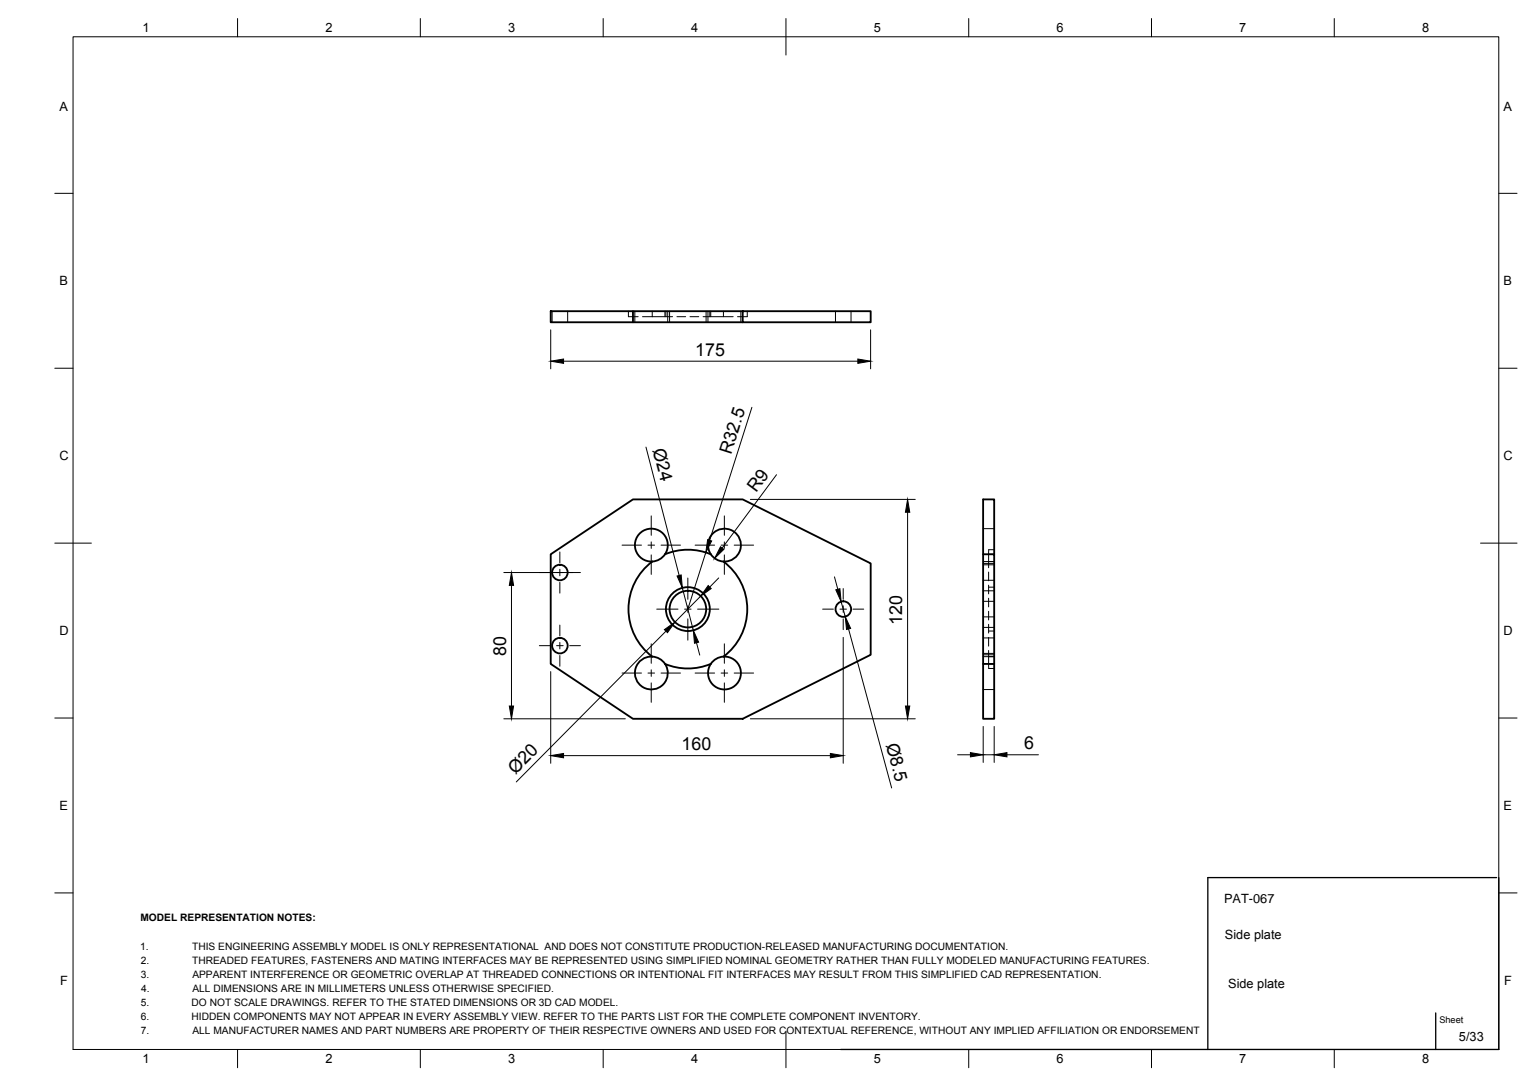
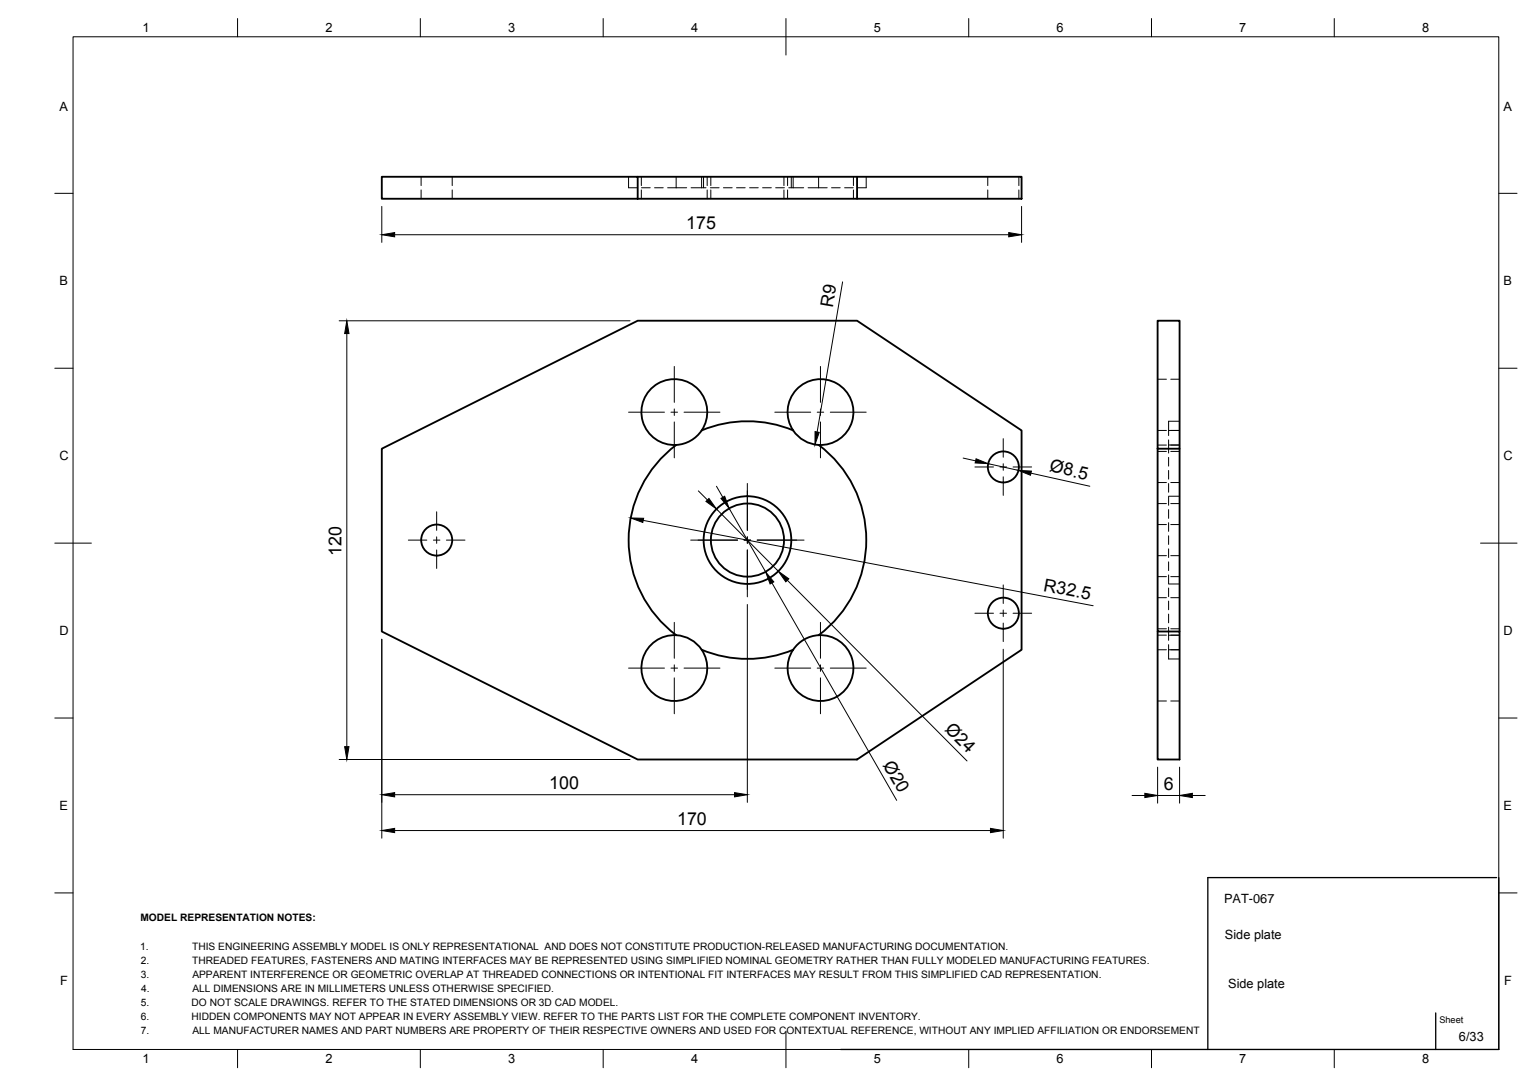
ISO-10303-21;
HEADER;
/* Generated by software containing ST-Developer
 * from STEP Tools, Inc. (www.steptools.com) 
 */

FILE_DESCRIPTION(
/* description */ ('Lifting hook block with sheave'),
/* implementation_level */ '2;1');

FILE_NAME(
/* name */ 'Side plate.step',
/* time_stamp */ '2026-10-28T03:23:54-07:00',
/* author */ (''),
/* organization */ (''),
/* preprocessor_version */ 'ST-DEVELOPER v20.2',
/* originating_system */ 'Autodesk Translation Framework v15.17.0.0',
/* authorisation */ '');

FILE_SCHEMA (('AUTOMOTIVE_DESIGN { 1 0 10303 214 3 1 1 }'));
ENDSEC;

DATA;
#10=MECHANICAL_DESIGN_GEOMETRIC_PRESENTATION_REPRESENTATION('',(#351),#9391);
#291=SHAPE_REPRESENTATION_RELATIONSHIP('SRR','None',#9522,#321);
#321=ADVANCED_BREP_SHAPE_REPRESENTATION('',(#389),#9357);
#351=STYLED_ITEM('',(#9752),#389);
#389=MANIFOLD_SOLID_BREP('Body1',#4887);
#424=LINE('',#7581,#712);
#425=LINE('',#7583,#713);
#426=LINE('',#7587,#714);
#427=LINE('',#7590,#715);
#428=LINE('',#7593,#716);
#429=LINE('',#7595,#717);
#430=LINE('',#7599,#718);
#431=LINE('',#7603,#719);
#432=LINE('',#7606,#720);
#433=LINE('',#7611,#721);
#434=LINE('',#7618,#722);
#435=LINE('',#7625,#723);
#436=LINE('',#7635,#724);
#437=LINE('',#7642,#725);
#438=LINE('',#7648,#726);
#439=LINE('',#7654,#727);
#440=LINE('',#7659,#728);
#441=LINE('',#7663,#729);
#442=LINE('',#7665,#730);
#443=LINE('',#7667,#731);
#444=LINE('',#7668,#732);
#445=LINE('',#7671,#733);
#446=LINE('',#7673,#734);
#447=LINE('',#7674,#735);
#448=LINE('',#7677,#736);
#449=LINE('',#7679,#737);
#450=LINE('',#7680,#738);
#451=LINE('',#7683,#739);
#452=LINE('',#7685,#740);
#453=LINE('',#7686,#741);
#454=LINE('',#7689,#742);
#455=LINE('',#7691,#743);
#456=LINE('',#7692,#744);
#457=LINE('',#7695,#745);
#458=LINE('',#7697,#746);
#459=LINE('',#7698,#747);
#460=LINE('',#7701,#748);
#461=LINE('',#7703,#749);
#462=LINE('',#7704,#750);
#463=LINE('',#7706,#751);
#464=LINE('',#7707,#752);
#712=VECTOR('',#5957,1.);
#713=VECTOR('',#5958,1.);
#714=VECTOR('',#5963,1.);
#715=VECTOR('',#5966,1.);
#716=VECTOR('',#5969,1.);
#717=VECTOR('',#5970,1.);
#718=VECTOR('',#5975,1.2);
#719=VECTOR('',#5980,1.);
#720=VECTOR('',#5983,1.);
#721=VECTOR('',#5988,0.9);
#722=VECTOR('',#5997,0.9);
#723=VECTOR('',#6006,0.9);
#724=VECTOR('',#6019,0.9);
#725=VECTOR('',#6028,0.425);
#726=VECTOR('',#6035,0.425);
#727=VECTOR('',#6042,0.425);
#728=VECTOR('',#6049,1.);
#729=VECTOR('',#6052,1.);
#730=VECTOR('',#6053,1.);
#731=VECTOR('',#6054,1.);
#732=VECTOR('',#6055,1.);
#733=VECTOR('',#6058,1.);
#734=VECTOR('',#6059,1.);
#735=VECTOR('',#6060,1.);
#736=VECTOR('',#6063,1.);
#737=VECTOR('',#6064,1.);
#738=VECTOR('',#6065,1.);
#739=VECTOR('',#6068,1.);
#740=VECTOR('',#6069,1.);
#741=VECTOR('',#6070,1.);
#742=VECTOR('',#6073,1.);
#743=VECTOR('',#6074,1.);
#744=VECTOR('',#6075,1.);
#745=VECTOR('',#6078,1.);
#746=VECTOR('',#6079,1.);
#747=VECTOR('',#6080,1.);
#748=VECTOR('',#6083,1.);
#749=VECTOR('',#6084,1.);
#750=VECTOR('',#6085,1.);
#751=VECTOR('',#6088,1.);
#752=VECTOR('',#6089,1.);
#1000=CYLINDRICAL_SURFACE('',#5272,3.25);
#1001=CYLINDRICAL_SURFACE('',#5274,3.25);
#1002=CYLINDRICAL_SURFACE('',#5276,3.25);
#1003=CYLINDRICAL_SURFACE('',#5278,1.2);
#1004=CYLINDRICAL_SURFACE('',#5280,3.25);
#1005=CYLINDRICAL_SURFACE('',#5282,0.9);
#1006=CYLINDRICAL_SURFACE('',#5286,0.9);
#1007=CYLINDRICAL_SURFACE('',#5290,0.9);
#1008=CYLINDRICAL_SURFACE('',#5296,0.9);
#1009=CYLINDRICAL_SURFACE('',#5300,0.425);
#1010=CYLINDRICAL_SURFACE('',#5303,0.425);
#1011=CYLINDRICAL_SURFACE('',#5306,0.425);
#1012=CYLINDRICAL_SURFACE('',#5309,1.);
#1107=FACE_BOUND('',#1512,.T.);
#1108=FACE_BOUND('',#1522,.T.);
#1109=FACE_BOUND('',#1537,.T.);
#1110=FACE_BOUND('',#1538,.T.);
#1111=FACE_BOUND('',#1539,.T.);
#1112=FACE_BOUND('',#1540,.T.);
#1113=FACE_BOUND('',#1542,.T.);
#1114=FACE_BOUND('',#1543,.T.);
#1115=FACE_BOUND('',#1544,.T.);
#1116=FACE_BOUND('',#1545,.T.);
#1117=FACE_BOUND('',#1546,.T.);
#1118=FACE_BOUND('',#1547,.T.);
#1119=FACE_BOUND('',#1548,.T.);
#1120=FACE_BOUND('',#1549,.T.);
#1222=FACE_OUTER_BOUND('',#1511,.T.);
#1223=FACE_OUTER_BOUND('',#1513,.T.);
#1224=FACE_OUTER_BOUND('',#1514,.T.);
#1225=FACE_OUTER_BOUND('',#1515,.T.);
#1226=FACE_OUTER_BOUND('',#1516,.T.);
#1227=FACE_OUTER_BOUND('',#1517,.T.);
#1228=FACE_OUTER_BOUND('',#1518,.T.);
#1229=FACE_OUTER_BOUND('',#1519,.T.);
#1230=FACE_OUTER_BOUND('',#1520,.T.);
#1231=FACE_OUTER_BOUND('',#1521,.T.);
#1232=FACE_OUTER_BOUND('',#1523,.T.);
#1233=FACE_OUTER_BOUND('',#1524,.T.);
#1234=FACE_OUTER_BOUND('',#1525,.T.);
#1235=FACE_OUTER_BOUND('',#1526,.T.);
#1236=FACE_OUTER_BOUND('',#1527,.T.);
#1237=FACE_OUTER_BOUND('',#1528,.T.);
#1238=FACE_OUTER_BOUND('',#1529,.T.);
#1239=FACE_OUTER_BOUND('',#1530,.T.);
#1240=FACE_OUTER_BOUND('',#1531,.T.);
#1241=FACE_OUTER_BOUND('',#1532,.T.);
#1242=FACE_OUTER_BOUND('',#1533,.T.);
#1243=FACE_OUTER_BOUND('',#1534,.T.);
#1244=FACE_OUTER_BOUND('',#1535,.T.);
#1245=FACE_OUTER_BOUND('',#1536,.T.);
#1246=FACE_OUTER_BOUND('',#1541,.T.);
#1511=EDGE_LOOP('',(#3230,#3231,#3232,#3233,#3234,#3235,#3236,#3237));
#1512=EDGE_LOOP('',(#3238));
#1513=EDGE_LOOP('',(#3239,#3240,#3241,#3242));
#1514=EDGE_LOOP('',(#3243,#3244,#3245,#3246));
#1515=EDGE_LOOP('',(#3247,#3248,#3249,#3250));
#1516=EDGE_LOOP('',(#3251,#3252,#3253,#3254));
#1517=EDGE_LOOP('',(#3255,#3256,#3257,#3258));
#1518=EDGE_LOOP('',(#3259,#3260,#3261,#3262,#3263,#3264,#3265,#3266));
#1519=EDGE_LOOP('',(#3267,#3268,#3269,#3270,#3271,#3272,#3273,#3274));
#1520=EDGE_LOOP('',(#3275,#3276,#3277,#3278,#3279,#3280,#3281,#3282));
#1521=EDGE_LOOP('',(#3283));
#1522=EDGE_LOOP('',(#3284));
#1523=EDGE_LOOP('',(#3285,#3286,#3287,#3288,#3289,#3290,#3291,#3292));
#1524=EDGE_LOOP('',(#3293,#3294,#3295,#3296));
#1525=EDGE_LOOP('',(#3297,#3298,#3299,#3300));
#1526=EDGE_LOOP('',(#3301,#3302,#3303,#3304));
#1527=EDGE_LOOP('',(#3305,#3306,#3307,#3308));
#1528=EDGE_LOOP('',(#3309,#3310,#3311,#3312));
#1529=EDGE_LOOP('',(#3313,#3314,#3315,#3316));
#1530=EDGE_LOOP('',(#3317,#3318,#3319,#3320));
#1531=EDGE_LOOP('',(#3321,#3322,#3323,#3324));
#1532=EDGE_LOOP('',(#3325,#3326,#3327,#3328));
#1533=EDGE_LOOP('',(#3329,#3330,#3331,#3332));
#1534=EDGE_LOOP('',(#3333,#3334,#3335,#3336));
#1535=EDGE_LOOP('',(#3337,#3338,#3339,#3340));
#1536=EDGE_LOOP('',(#3341,#3342,#3343,#3344,#3345,#3346,#3347,#3348));
#1537=EDGE_LOOP('',(#3349,#3350,#3351,#3352,#3353,#3354,#3355,#3356,#3357,
#3358,#3359,#3360));
#1538=EDGE_LOOP('',(#3361));
#1539=EDGE_LOOP('',(#3362));
#1540=EDGE_LOOP('',(#3363));
#1541=EDGE_LOOP('',(#3364,#3365,#3366,#3367,#3368,#3369,#3370,#3371));
#1542=EDGE_LOOP('',(#3372));
#1543=EDGE_LOOP('',(#3373));
#1544=EDGE_LOOP('',(#3374));
#1545=EDGE_LOOP('',(#3375));
#1546=EDGE_LOOP('',(#3376));
#1547=EDGE_LOOP('',(#3377));
#1548=EDGE_LOOP('',(#3378));
#1549=EDGE_LOOP('',(#3379));
#1915=CIRCLE('',#5263,0.9);
#1916=CIRCLE('',#5264,3.25);
#1917=CIRCLE('',#5265,0.9);
#1918=CIRCLE('',#5266,3.25);
#1919=CIRCLE('',#5267,0.9);
#1920=CIRCLE('',#5268,3.25);
#1921=CIRCLE('',#5269,0.9);
#1922=CIRCLE('',#5270,3.25);
#1923=CIRCLE('',#5271,1.2);
#1924=CIRCLE('',#5273,3.25);
#1925=CIRCLE('',#5275,3.25);
#1926=CIRCLE('',#5277,3.25);
#1927=CIRCLE('',#5279,1.2);
#1928=CIRCLE('',#5281,3.25);
#1929=CIRCLE('',#5283,0.9);
#1930=CIRCLE('',#5284,0.9);
#1931=CIRCLE('',#5285,0.9);
#1932=CIRCLE('',#5287,0.9);
#1933=CIRCLE('',#5288,0.9);
#1934=CIRCLE('',#5289,0.9);
#1935=CIRCLE('',#5291,0.9);
#1936=CIRCLE('',#5292,0.9);
#1937=CIRCLE('',#5293,0.9);
#1938=CIRCLE('',#5295,1.);
#1939=CIRCLE('',#5297,0.9);
#1940=CIRCLE('',#5298,0.9);
#1941=CIRCLE('',#5299,0.9);
#1942=CIRCLE('',#5301,0.425);
#1943=CIRCLE('',#5302,0.425);
#1944=CIRCLE('',#5304,0.425);
#1945=CIRCLE('',#5305,0.425);
#1946=CIRCLE('',#5307,0.425);
#1947=CIRCLE('',#5308,0.425);
#1948=CIRCLE('',#5310,1.);
#2208=VERTEX_POINT('',#7561);
#2209=VERTEX_POINT('',#7562);
#2210=VERTEX_POINT('',#7564);
#2211=VERTEX_POINT('',#7566);
#2212=VERTEX_POINT('',#7568);
#2213=VERTEX_POINT('',#7570);
#2214=VERTEX_POINT('',#7572);
#2215=VERTEX_POINT('',#7574);
#2216=VERTEX_POINT('',#7577);
#2217=VERTEX_POINT('',#7580);
#2218=VERTEX_POINT('',#7582);
#2219=VERTEX_POINT('',#7586);
#2220=VERTEX_POINT('',#7588);
#2221=VERTEX_POINT('',#7592);
#2222=VERTEX_POINT('',#7594);
#2223=VERTEX_POINT('',#7598);
#2224=VERTEX_POINT('',#7602);
#2225=VERTEX_POINT('',#7604);
#2226=VERTEX_POINT('',#7608);
#2227=VERTEX_POINT('',#7610);
#2228=VERTEX_POINT('',#7615);
#2229=VERTEX_POINT('',#7617);
#2230=VERTEX_POINT('',#7622);
#2231=VERTEX_POINT('',#7624);
#2232=VERTEX_POINT('',#7629);
#2233=VERTEX_POINT('',#7632);
#2234=VERTEX_POINT('',#7634);
#2235=VERTEX_POINT('',#7639);
#2236=VERTEX_POINT('',#7641);
#2237=VERTEX_POINT('',#7645);
#2238=VERTEX_POINT('',#7647);
#2239=VERTEX_POINT('',#7651);
#2240=VERTEX_POINT('',#7653);
#2241=VERTEX_POINT('',#7657);
#2242=VERTEX_POINT('',#7661);
#2243=VERTEX_POINT('',#7662);
#2244=VERTEX_POINT('',#7664);
#2245=VERTEX_POINT('',#7666);
#2246=VERTEX_POINT('',#7670);
#2247=VERTEX_POINT('',#7672);
#2248=VERTEX_POINT('',#7676);
#2249=VERTEX_POINT('',#7678);
#2250=VERTEX_POINT('',#7682);
#2251=VERTEX_POINT('',#7684);
#2252=VERTEX_POINT('',#7688);
#2253=VERTEX_POINT('',#7690);
#2254=VERTEX_POINT('',#7694);
#2255=VERTEX_POINT('',#7696);
#2256=VERTEX_POINT('',#7700);
#2257=VERTEX_POINT('',#7702);
#2619=EDGE_CURVE('',#2208,#2209,#1915,.T.);
#2620=EDGE_CURVE('',#2208,#2210,#1916,.T.);
#2621=EDGE_CURVE('',#2211,#2210,#1917,.T.);
#2622=EDGE_CURVE('',#2211,#2212,#1918,.T.);
#2623=EDGE_CURVE('',#2213,#2212,#1919,.T.);
#2624=EDGE_CURVE('',#2213,#2214,#1920,.T.);
#2625=EDGE_CURVE('',#2215,#2214,#1921,.T.);
#2626=EDGE_CURVE('',#2215,#2209,#1922,.T.);
#2627=EDGE_CURVE('',#2216,#2216,#1923,.T.);
#2628=EDGE_CURVE('',#2214,#2217,#424,.T.);
#2629=EDGE_CURVE('',#2218,#2213,#425,.T.);
#2630=EDGE_CURVE('',#2217,#2218,#1924,.T.);
#2631=EDGE_CURVE('',#2219,#2211,#426,.T.);
#2632=EDGE_CURVE('',#2220,#2219,#1925,.T.);
#2633=EDGE_CURVE('',#2212,#2220,#427,.T.);
#2634=EDGE_CURVE('',#2209,#2221,#428,.T.);
#2635=EDGE_CURVE('',#2222,#2215,#429,.T.);
#2636=EDGE_CURVE('',#2221,#2222,#1926,.T.);
#2637=EDGE_CURVE('',#2216,#2223,#430,.T.);
#2638=EDGE_CURVE('',#2223,#2223,#1927,.T.);
#2639=EDGE_CURVE('',#2224,#2208,#431,.T.);
#2640=EDGE_CURVE('',#2225,#2224,#1928,.T.);
#2641=EDGE_CURVE('',#2210,#2225,#432,.T.);
#2642=EDGE_CURVE('',#2226,#2226,#1929,.T.);
#2643=EDGE_CURVE('',#2226,#2227,#433,.T.);
#2644=EDGE_CURVE('',#2224,#2227,#1930,.T.);
#2645=EDGE_CURVE('',#2227,#2221,#1931,.T.);
#2646=EDGE_CURVE('',#2228,#2228,#1932,.T.);
#2647=EDGE_CURVE('',#2228,#2229,#434,.T.);
#2648=EDGE_CURVE('',#2222,#2229,#1933,.T.);
#2649=EDGE_CURVE('',#2229,#2217,#1934,.T.);
#2650=EDGE_CURVE('',#2230,#2230,#1935,.T.);
#2651=EDGE_CURVE('',#2230,#2231,#435,.T.);
#2652=EDGE_CURVE('',#2218,#2231,#1936,.T.);
#2653=EDGE_CURVE('',#2231,#2220,#1937,.T.);
#2654=EDGE_CURVE('',#2232,#2232,#1938,.T.);
#2655=EDGE_CURVE('',#2233,#2233,#1939,.T.);
#2656=EDGE_CURVE('',#2233,#2234,#436,.T.);
#2657=EDGE_CURVE('',#2219,#2234,#1940,.T.);
#2658=EDGE_CURVE('',#2234,#2225,#1941,.T.);
#2659=EDGE_CURVE('',#2235,#2235,#1942,.T.);
#2660=EDGE_CURVE('',#2235,#2236,#437,.T.);
#2661=EDGE_CURVE('',#2236,#2236,#1943,.T.);
#2662=EDGE_CURVE('',#2237,#2237,#1944,.T.);
#2663=EDGE_CURVE('',#2237,#2238,#438,.T.);
#2664=EDGE_CURVE('',#2238,#2238,#1945,.T.);
#2665=EDGE_CURVE('',#2239,#2239,#1946,.T.);
#2666=EDGE_CURVE('',#2239,#2240,#439,.T.);
#2667=EDGE_CURVE('',#2240,#2240,#1947,.T.);
#2668=EDGE_CURVE('',#2241,#2241,#1948,.T.);
#2669=EDGE_CURVE('',#2241,#2232,#440,.T.);
#2670=EDGE_CURVE('',#2242,#2243,#441,.T.);
#2671=EDGE_CURVE('',#2242,#2244,#442,.T.);
#2672=EDGE_CURVE('',#2245,#2244,#443,.T.);
#2673=EDGE_CURVE('',#2243,#2245,#444,.T.);
#2674=EDGE_CURVE('',#2243,#2246,#445,.T.);
#2675=EDGE_CURVE('',#2247,#2245,#446,.T.);
#2676=EDGE_CURVE('',#2246,#2247,#447,.T.);
#2677=EDGE_CURVE('',#2246,#2248,#448,.T.);
#2678=EDGE_CURVE('',#2249,#2247,#449,.T.);
#2679=EDGE_CURVE('',#2248,#2249,#450,.T.);
#2680=EDGE_CURVE('',#2248,#2250,#451,.T.);
#2681=EDGE_CURVE('',#2251,#2249,#452,.T.);
#2682=EDGE_CURVE('',#2250,#2251,#453,.T.);
#2683=EDGE_CURVE('',#2250,#2252,#454,.T.);
#2684=EDGE_CURVE('',#2253,#2251,#455,.T.);
#2685=EDGE_CURVE('',#2252,#2253,#456,.T.);
#2686=EDGE_CURVE('',#2252,#2254,#457,.T.);
#2687=EDGE_CURVE('',#2255,#2253,#458,.T.);
#2688=EDGE_CURVE('',#2254,#2255,#459,.T.);
#2689=EDGE_CURVE('',#2254,#2256,#460,.T.);
#2690=EDGE_CURVE('',#2257,#2255,#461,.T.);
#2691=EDGE_CURVE('',#2256,#2257,#462,.T.);
#2692=EDGE_CURVE('',#2256,#2242,#463,.T.);
#2693=EDGE_CURVE('',#2244,#2257,#464,.T.);
#3230=ORIENTED_EDGE('',*,*,#2619,.F.);
#3231=ORIENTED_EDGE('',*,*,#2620,.T.);
#3232=ORIENTED_EDGE('',*,*,#2621,.F.);
#3233=ORIENTED_EDGE('',*,*,#2622,.T.);
#3234=ORIENTED_EDGE('',*,*,#2623,.F.);
#3235=ORIENTED_EDGE('',*,*,#2624,.T.);
#3236=ORIENTED_EDGE('',*,*,#2625,.F.);
#3237=ORIENTED_EDGE('',*,*,#2626,.T.);
#3238=ORIENTED_EDGE('',*,*,#2627,.T.);
#3239=ORIENTED_EDGE('',*,*,#2628,.F.);
#3240=ORIENTED_EDGE('',*,*,#2624,.F.);
#3241=ORIENTED_EDGE('',*,*,#2629,.F.);
#3242=ORIENTED_EDGE('',*,*,#2630,.F.);
#3243=ORIENTED_EDGE('',*,*,#2631,.F.);
#3244=ORIENTED_EDGE('',*,*,#2632,.F.);
#3245=ORIENTED_EDGE('',*,*,#2633,.F.);
#3246=ORIENTED_EDGE('',*,*,#2622,.F.);
#3247=ORIENTED_EDGE('',*,*,#2634,.F.);
#3248=ORIENTED_EDGE('',*,*,#2626,.F.);
#3249=ORIENTED_EDGE('',*,*,#2635,.F.);
#3250=ORIENTED_EDGE('',*,*,#2636,.F.);
#3251=ORIENTED_EDGE('',*,*,#2627,.F.);
#3252=ORIENTED_EDGE('',*,*,#2637,.T.);
#3253=ORIENTED_EDGE('',*,*,#2638,.F.);
#3254=ORIENTED_EDGE('',*,*,#2637,.F.);
#3255=ORIENTED_EDGE('',*,*,#2639,.F.);
#3256=ORIENTED_EDGE('',*,*,#2640,.F.);
#3257=ORIENTED_EDGE('',*,*,#2641,.F.);
#3258=ORIENTED_EDGE('',*,*,#2620,.F.);
#3259=ORIENTED_EDGE('',*,*,#2642,.F.);
#3260=ORIENTED_EDGE('',*,*,#2643,.T.);
#3261=ORIENTED_EDGE('',*,*,#2644,.F.);
#3262=ORIENTED_EDGE('',*,*,#2639,.T.);
#3263=ORIENTED_EDGE('',*,*,#2619,.T.);
#3264=ORIENTED_EDGE('',*,*,#2634,.T.);
#3265=ORIENTED_EDGE('',*,*,#2645,.F.);
#3266=ORIENTED_EDGE('',*,*,#2643,.F.);
#3267=ORIENTED_EDGE('',*,*,#2646,.F.);
#3268=ORIENTED_EDGE('',*,*,#2647,.T.);
#3269=ORIENTED_EDGE('',*,*,#2648,.F.);
#3270=ORIENTED_EDGE('',*,*,#2635,.T.);
#3271=ORIENTED_EDGE('',*,*,#2625,.T.);
#3272=ORIENTED_EDGE('',*,*,#2628,.T.);
#3273=ORIENTED_EDGE('',*,*,#2649,.F.);
#3274=ORIENTED_EDGE('',*,*,#2647,.F.);
#3275=ORIENTED_EDGE('',*,*,#2650,.F.);
#3276=ORIENTED_EDGE('',*,*,#2651,.T.);
#3277=ORIENTED_EDGE('',*,*,#2652,.F.);
#3278=ORIENTED_EDGE('',*,*,#2629,.T.);
#3279=ORIENTED_EDGE('',*,*,#2623,.T.);
#3280=ORIENTED_EDGE('',*,*,#2633,.T.);
#3281=ORIENTED_EDGE('',*,*,#2653,.F.);
#3282=ORIENTED_EDGE('',*,*,#2651,.F.);
#3283=ORIENTED_EDGE('',*,*,#2638,.T.);
#3284=ORIENTED_EDGE('',*,*,#2654,.T.);
#3285=ORIENTED_EDGE('',*,*,#2655,.F.);
#3286=ORIENTED_EDGE('',*,*,#2656,.T.);
#3287=ORIENTED_EDGE('',*,*,#2657,.F.);
#3288=ORIENTED_EDGE('',*,*,#2631,.T.);
#3289=ORIENTED_EDGE('',*,*,#2621,.T.);
#3290=ORIENTED_EDGE('',*,*,#2641,.T.);
#3291=ORIENTED_EDGE('',*,*,#2658,.F.);
#3292=ORIENTED_EDGE('',*,*,#2656,.F.);
#3293=ORIENTED_EDGE('',*,*,#2659,.F.);
#3294=ORIENTED_EDGE('',*,*,#2660,.T.);
#3295=ORIENTED_EDGE('',*,*,#2661,.F.);
#3296=ORIENTED_EDGE('',*,*,#2660,.F.);
#3297=ORIENTED_EDGE('',*,*,#2662,.F.);
#3298=ORIENTED_EDGE('',*,*,#2663,.T.);
#3299=ORIENTED_EDGE('',*,*,#2664,.F.);
#3300=ORIENTED_EDGE('',*,*,#2663,.F.);
#3301=ORIENTED_EDGE('',*,*,#2665,.F.);
#3302=ORIENTED_EDGE('',*,*,#2666,.T.);
#3303=ORIENTED_EDGE('',*,*,#2667,.F.);
#3304=ORIENTED_EDGE('',*,*,#2666,.F.);
#3305=ORIENTED_EDGE('',*,*,#2668,.F.);
#3306=ORIENTED_EDGE('',*,*,#2669,.T.);
#3307=ORIENTED_EDGE('',*,*,#2654,.F.);
#3308=ORIENTED_EDGE('',*,*,#2669,.F.);
#3309=ORIENTED_EDGE('',*,*,#2670,.F.);
#3310=ORIENTED_EDGE('',*,*,#2671,.T.);
#3311=ORIENTED_EDGE('',*,*,#2672,.F.);
#3312=ORIENTED_EDGE('',*,*,#2673,.F.);
#3313=ORIENTED_EDGE('',*,*,#2674,.F.);
#3314=ORIENTED_EDGE('',*,*,#2673,.T.);
#3315=ORIENTED_EDGE('',*,*,#2675,.F.);
#3316=ORIENTED_EDGE('',*,*,#2676,.F.);
#3317=ORIENTED_EDGE('',*,*,#2677,.F.);
#3318=ORIENTED_EDGE('',*,*,#2676,.T.);
#3319=ORIENTED_EDGE('',*,*,#2678,.F.);
#3320=ORIENTED_EDGE('',*,*,#2679,.F.);
#3321=ORIENTED_EDGE('',*,*,#2680,.F.);
#3322=ORIENTED_EDGE('',*,*,#2679,.T.);
#3323=ORIENTED_EDGE('',*,*,#2681,.F.);
#3324=ORIENTED_EDGE('',*,*,#2682,.F.);
#3325=ORIENTED_EDGE('',*,*,#2683,.F.);
#3326=ORIENTED_EDGE('',*,*,#2682,.T.);
#3327=ORIENTED_EDGE('',*,*,#2684,.F.);
#3328=ORIENTED_EDGE('',*,*,#2685,.F.);
#3329=ORIENTED_EDGE('',*,*,#2686,.F.);
#3330=ORIENTED_EDGE('',*,*,#2685,.T.);
#3331=ORIENTED_EDGE('',*,*,#2687,.F.);
#3332=ORIENTED_EDGE('',*,*,#2688,.F.);
#3333=ORIENTED_EDGE('',*,*,#2689,.F.);
#3334=ORIENTED_EDGE('',*,*,#2688,.T.);
#3335=ORIENTED_EDGE('',*,*,#2690,.F.);
#3336=ORIENTED_EDGE('',*,*,#2691,.F.);
#3337=ORIENTED_EDGE('',*,*,#2692,.F.);
#3338=ORIENTED_EDGE('',*,*,#2691,.T.);
#3339=ORIENTED_EDGE('',*,*,#2693,.F.);
#3340=ORIENTED_EDGE('',*,*,#2671,.F.);
#3341=ORIENTED_EDGE('',*,*,#2693,.T.);
#3342=ORIENTED_EDGE('',*,*,#2690,.T.);
#3343=ORIENTED_EDGE('',*,*,#2687,.T.);
#3344=ORIENTED_EDGE('',*,*,#2684,.T.);
#3345=ORIENTED_EDGE('',*,*,#2681,.T.);
#3346=ORIENTED_EDGE('',*,*,#2678,.T.);
#3347=ORIENTED_EDGE('',*,*,#2675,.T.);
#3348=ORIENTED_EDGE('',*,*,#2672,.T.);
#3349=ORIENTED_EDGE('',*,*,#2640,.T.);
#3350=ORIENTED_EDGE('',*,*,#2644,.T.);
#3351=ORIENTED_EDGE('',*,*,#2645,.T.);
#3352=ORIENTED_EDGE('',*,*,#2636,.T.);
#3353=ORIENTED_EDGE('',*,*,#2648,.T.);
#3354=ORIENTED_EDGE('',*,*,#2649,.T.);
#3355=ORIENTED_EDGE('',*,*,#2630,.T.);
#3356=ORIENTED_EDGE('',*,*,#2652,.T.);
#3357=ORIENTED_EDGE('',*,*,#2653,.T.);
#3358=ORIENTED_EDGE('',*,*,#2632,.T.);
#3359=ORIENTED_EDGE('',*,*,#2657,.T.);
#3360=ORIENTED_EDGE('',*,*,#2658,.T.);
#3361=ORIENTED_EDGE('',*,*,#2667,.T.);
#3362=ORIENTED_EDGE('',*,*,#2664,.T.);
#3363=ORIENTED_EDGE('',*,*,#2661,.T.);
#3364=ORIENTED_EDGE('',*,*,#2692,.T.);
#3365=ORIENTED_EDGE('',*,*,#2670,.T.);
#3366=ORIENTED_EDGE('',*,*,#2674,.T.);
#3367=ORIENTED_EDGE('',*,*,#2677,.T.);
#3368=ORIENTED_EDGE('',*,*,#2680,.T.);
#3369=ORIENTED_EDGE('',*,*,#2683,.T.);
#3370=ORIENTED_EDGE('',*,*,#2686,.T.);
#3371=ORIENTED_EDGE('',*,*,#2689,.T.);
#3372=ORIENTED_EDGE('',*,*,#2668,.T.);
#3373=ORIENTED_EDGE('',*,*,#2665,.T.);
#3374=ORIENTED_EDGE('',*,*,#2662,.T.);
#3375=ORIENTED_EDGE('',*,*,#2659,.T.);
#3376=ORIENTED_EDGE('',*,*,#2650,.T.);
#3377=ORIENTED_EDGE('',*,*,#2642,.T.);
#3378=ORIENTED_EDGE('',*,*,#2655,.T.);
#3379=ORIENTED_EDGE('',*,*,#2646,.T.);
#4452=PLANE('',#5262);
#4453=PLANE('',#5294);
#4454=PLANE('',#5311);
#4455=PLANE('',#5312);
#4456=PLANE('',#5313);
#4457=PLANE('',#5314);
#4458=PLANE('',#5315);
#4459=PLANE('',#5316);
#4460=PLANE('',#5317);
#4461=PLANE('',#5318);
#4462=PLANE('',#5319);
#4463=PLANE('',#5320);
#4598=ADVANCED_FACE('',(#1222,#1107),#4452,.T.);
#4599=ADVANCED_FACE('',(#1223),#1000,.F.);
#4600=ADVANCED_FACE('',(#1224),#1001,.F.);
#4601=ADVANCED_FACE('',(#1225),#1002,.F.);
#4602=ADVANCED_FACE('',(#1226),#1003,.T.);
#4603=ADVANCED_FACE('',(#1227),#1004,.F.);
#4604=ADVANCED_FACE('',(#1228),#1005,.F.);
#4605=ADVANCED_FACE('',(#1229),#1006,.F.);
#4606=ADVANCED_FACE('',(#1230),#1007,.F.);
#4607=ADVANCED_FACE('',(#1231,#1108),#4453,.T.);
#4608=ADVANCED_FACE('',(#1232),#1008,.F.);
#4609=ADVANCED_FACE('',(#1233),#1009,.F.);
#4610=ADVANCED_FACE('',(#1234),#1010,.F.);
#4611=ADVANCED_FACE('',(#1235),#1011,.F.);
#4612=ADVANCED_FACE('',(#1236),#1012,.F.);
#4613=ADVANCED_FACE('',(#1237),#4454,.T.);
#4614=ADVANCED_FACE('',(#1238),#4455,.T.);
#4615=ADVANCED_FACE('',(#1239),#4456,.T.);
#4616=ADVANCED_FACE('',(#1240),#4457,.T.);
#4617=ADVANCED_FACE('',(#1241),#4458,.T.);
#4618=ADVANCED_FACE('',(#1242),#4459,.T.);
#4619=ADVANCED_FACE('',(#1243),#4460,.T.);
#4620=ADVANCED_FACE('',(#1244),#4461,.T.);
#4621=ADVANCED_FACE('',(#1245,#1109,#1110,#1111,#1112),#4462,.T.);
#4622=ADVANCED_FACE('',(#1246,#1113,#1114,#1115,#1116,#1117,#1118,#1119,
#1120),#4463,.F.);
#4887=CLOSED_SHELL('',(#4598,#4599,#4600,#4601,#4602,#4603,#4604,#4605,
#4606,#4607,#4608,#4609,#4610,#4611,#4612,#4613,#4614,#4615,#4616,#4617,
#4618,#4619,#4620,#4621,#4622));
#5261=AXIS2_PLACEMENT_3D('',#7559,#5933,#5934);
#5262=AXIS2_PLACEMENT_3D('',#7560,#5935,#5936);
#5263=AXIS2_PLACEMENT_3D('',#7563,#5937,#5938);
#5264=AXIS2_PLACEMENT_3D('',#7565,#5939,#5940);
#5265=AXIS2_PLACEMENT_3D('',#7567,#5941,#5942);
#5266=AXIS2_PLACEMENT_3D('',#7569,#5943,#5944);
#5267=AXIS2_PLACEMENT_3D('',#7571,#5945,#5946);
#5268=AXIS2_PLACEMENT_3D('',#7573,#5947,#5948);
#5269=AXIS2_PLACEMENT_3D('',#7575,#5949,#5950);
#5270=AXIS2_PLACEMENT_3D('',#7576,#5951,#5952);
#5271=AXIS2_PLACEMENT_3D('',#7578,#5953,#5954);
#5272=AXIS2_PLACEMENT_3D('',#7579,#5955,#5956);
#5273=AXIS2_PLACEMENT_3D('',#7584,#5959,#5960);
#5274=AXIS2_PLACEMENT_3D('',#7585,#5961,#5962);
#5275=AXIS2_PLACEMENT_3D('',#7589,#5964,#5965);
#5276=AXIS2_PLACEMENT_3D('',#7591,#5967,#5968);
#5277=AXIS2_PLACEMENT_3D('',#7596,#5971,#5972);
#5278=AXIS2_PLACEMENT_3D('',#7597,#5973,#5974);
#5279=AXIS2_PLACEMENT_3D('',#7600,#5976,#5977);
#5280=AXIS2_PLACEMENT_3D('',#7601,#5978,#5979);
#5281=AXIS2_PLACEMENT_3D('',#7605,#5981,#5982);
#5282=AXIS2_PLACEMENT_3D('',#7607,#5984,#5985);
#5283=AXIS2_PLACEMENT_3D('',#7609,#5986,#5987);
#5284=AXIS2_PLACEMENT_3D('',#7612,#5989,#5990);
#5285=AXIS2_PLACEMENT_3D('',#7613,#5991,#5992);
#5286=AXIS2_PLACEMENT_3D('',#7614,#5993,#5994);
#5287=AXIS2_PLACEMENT_3D('',#7616,#5995,#5996);
#5288=AXIS2_PLACEMENT_3D('',#7619,#5998,#5999);
#5289=AXIS2_PLACEMENT_3D('',#7620,#6000,#6001);
#5290=AXIS2_PLACEMENT_3D('',#7621,#6002,#6003);
#5291=AXIS2_PLACEMENT_3D('',#7623,#6004,#6005);
#5292=AXIS2_PLACEMENT_3D('',#7626,#6007,#6008);
#5293=AXIS2_PLACEMENT_3D('',#7627,#6009,#6010);
#5294=AXIS2_PLACEMENT_3D('',#7628,#6011,#6012);
#5295=AXIS2_PLACEMENT_3D('',#7630,#6013,#6014);
#5296=AXIS2_PLACEMENT_3D('',#7631,#6015,#6016);
#5297=AXIS2_PLACEMENT_3D('',#7633,#6017,#6018);
#5298=AXIS2_PLACEMENT_3D('',#7636,#6020,#6021);
#5299=AXIS2_PLACEMENT_3D('',#7637,#6022,#6023);
#5300=AXIS2_PLACEMENT_3D('',#7638,#6024,#6025);
#5301=AXIS2_PLACEMENT_3D('',#7640,#6026,#6027);
#5302=AXIS2_PLACEMENT_3D('',#7643,#6029,#6030);
#5303=AXIS2_PLACEMENT_3D('',#7644,#6031,#6032);
#5304=AXIS2_PLACEMENT_3D('',#7646,#6033,#6034);
#5305=AXIS2_PLACEMENT_3D('',#7649,#6036,#6037);
#5306=AXIS2_PLACEMENT_3D('',#7650,#6038,#6039);
#5307=AXIS2_PLACEMENT_3D('',#7652,#6040,#6041);
#5308=AXIS2_PLACEMENT_3D('',#7655,#6043,#6044);
#5309=AXIS2_PLACEMENT_3D('',#7656,#6045,#6046);
#5310=AXIS2_PLACEMENT_3D('',#7658,#6047,#6048);
#5311=AXIS2_PLACEMENT_3D('',#7660,#6050,#6051);
#5312=AXIS2_PLACEMENT_3D('',#7669,#6056,#6057);
#5313=AXIS2_PLACEMENT_3D('',#7675,#6061,#6062);
#5314=AXIS2_PLACEMENT_3D('',#7681,#6066,#6067);
#5315=AXIS2_PLACEMENT_3D('',#7687,#6071,#6072);
#5316=AXIS2_PLACEMENT_3D('',#7693,#6076,#6077);
#5317=AXIS2_PLACEMENT_3D('',#7699,#6081,#6082);
#5318=AXIS2_PLACEMENT_3D('',#7705,#6086,#6087);
#5319=AXIS2_PLACEMENT_3D('',#7708,#6090,#6091);
#5320=AXIS2_PLACEMENT_3D('',#7709,#6092,#6093);
#5933=DIRECTION('axis',(0.,0.,1.));
#5934=DIRECTION('refdir',(1.,0.,0.));
#5935=DIRECTION('center_axis',(0.,1.,0.));
#5936=DIRECTION('ref_axis',(1.,0.,0.));
#5937=DIRECTION('center_axis',(0.,1.,0.));
#5938=DIRECTION('ref_axis',(1.,0.,0.));
#5939=DIRECTION('center_axis',(0.,1.,0.));
#5940=DIRECTION('ref_axis',(1.,0.,0.));
#5941=DIRECTION('center_axis',(0.,1.,0.));
#5942=DIRECTION('ref_axis',(1.,0.,0.));
#5943=DIRECTION('center_axis',(0.,1.,0.));
#5944=DIRECTION('ref_axis',(1.,0.,0.));
#5945=DIRECTION('center_axis',(0.,1.,0.));
#5946=DIRECTION('ref_axis',(1.,0.,0.));
#5947=DIRECTION('center_axis',(0.,1.,0.));
#5948=DIRECTION('ref_axis',(1.,0.,0.));
#5949=DIRECTION('center_axis',(0.,1.,0.));
#5950=DIRECTION('ref_axis',(1.,0.,0.));
#5951=DIRECTION('center_axis',(0.,1.,0.));
#5952=DIRECTION('ref_axis',(1.,0.,0.));
#5953=DIRECTION('center_axis',(0.,-1.,0.));
#5954=DIRECTION('ref_axis',(1.,0.,0.));
#5955=DIRECTION('center_axis',(0.,1.,0.));
#5956=DIRECTION('ref_axis',(1.,0.,0.));
#5957=DIRECTION('',(0.,1.,0.));
#5958=DIRECTION('',(0.,-1.,0.));
#5959=DIRECTION('center_axis',(0.,-1.,0.));
#5960=DIRECTION('ref_axis',(1.,0.,0.));
#5961=DIRECTION('center_axis',(0.,1.,0.));
#5962=DIRECTION('ref_axis',(1.,0.,0.));
#5963=DIRECTION('',(0.,-1.,0.));
#5964=DIRECTION('center_axis',(0.,-1.,0.));
#5965=DIRECTION('ref_axis',(1.,0.,0.));
#5966=DIRECTION('',(0.,1.,0.));
#5967=DIRECTION('center_axis',(0.,1.,0.));
#5968=DIRECTION('ref_axis',(1.,0.,0.));
#5969=DIRECTION('',(0.,1.,0.));
#5970=DIRECTION('',(0.,-1.,0.));
#5971=DIRECTION('center_axis',(0.,-1.,0.));
#5972=DIRECTION('ref_axis',(1.,0.,0.));
#5973=DIRECTION('center_axis',(0.,1.,0.));
#5974=DIRECTION('ref_axis',(1.,0.,0.));
#5975=DIRECTION('',(0.,1.,0.));
#5976=DIRECTION('center_axis',(0.,1.,0.));
#5977=DIRECTION('ref_axis',(1.,0.,0.));
#5978=DIRECTION('center_axis',(0.,1.,0.));
#5979=DIRECTION('ref_axis',(-1.,0.,-1.22464679914735E-16));
#5980=DIRECTION('',(0.,-1.,0.));
#5981=DIRECTION('center_axis',(0.,-1.,0.));
#5982=DIRECTION('ref_axis',(1.,0.,0.));
#5983=DIRECTION('',(0.,1.,0.));
#5984=DIRECTION('center_axis',(0.,1.,0.));
#5985=DIRECTION('ref_axis',(1.,0.,0.));
#5986=DIRECTION('center_axis',(0.,1.,0.));
#5987=DIRECTION('ref_axis',(1.,0.,0.));
#5988=DIRECTION('',(0.,1.,0.));
#5989=DIRECTION('center_axis',(0.,-1.,0.));
#5990=DIRECTION('ref_axis',(1.,0.,0.));
#5991=DIRECTION('center_axis',(0.,-1.,0.));
#5992=DIRECTION('ref_axis',(1.,0.,0.));
#5993=DIRECTION('center_axis',(0.,1.,0.));
#5994=DIRECTION('ref_axis',(1.,0.,0.));
#5995=DIRECTION('center_axis',(0.,1.,0.));
#5996=DIRECTION('ref_axis',(1.,0.,0.));
#5997=DIRECTION('',(0.,1.,0.));
#5998=DIRECTION('center_axis',(0.,-1.,0.));
#5999=DIRECTION('ref_axis',(1.,0.,0.));
#6000=DIRECTION('center_axis',(0.,-1.,0.));
#6001=DIRECTION('ref_axis',(1.,0.,0.));
#6002=DIRECTION('center_axis',(0.,1.,0.));
#6003=DIRECTION('ref_axis',(1.,0.,0.));
#6004=DIRECTION('center_axis',(0.,1.,0.));
#6005=DIRECTION('ref_axis',(1.,0.,0.));
#6006=DIRECTION('',(0.,1.,0.));
#6007=DIRECTION('center_axis',(0.,-1.,0.));
#6008=DIRECTION('ref_axis',(1.,0.,0.));
#6009=DIRECTION('center_axis',(0.,-1.,0.));
#6010=DIRECTION('ref_axis',(1.,0.,0.));
#6011=DIRECTION('center_axis',(0.,1.,0.));
#6012=DIRECTION('ref_axis',(0.,0.,1.));
#6013=DIRECTION('center_axis',(0.,-1.,0.));
#6014=DIRECTION('ref_axis',(1.,0.,0.));
#6015=DIRECTION('center_axis',(0.,1.,0.));
#6016=DIRECTION('ref_axis',(1.,0.,0.));
#6017=DIRECTION('center_axis',(0.,1.,0.));
#6018=DIRECTION('ref_axis',(1.,0.,0.));
#6019=DIRECTION('',(0.,1.,0.));
#6020=DIRECTION('center_axis',(0.,-1.,0.));
#6021=DIRECTION('ref_axis',(1.,0.,0.));
#6022=DIRECTION('center_axis',(0.,-1.,0.));
#6023=DIRECTION('ref_axis',(1.,0.,0.));
#6024=DIRECTION('center_axis',(0.,1.,0.));
#6025=DIRECTION('ref_axis',(1.,0.,0.));
#6026=DIRECTION('center_axis',(0.,1.,0.));
#6027=DIRECTION('ref_axis',(1.,0.,0.));
#6028=DIRECTION('',(0.,1.,0.));
#6029=DIRECTION('center_axis',(0.,-1.,0.));
#6030=DIRECTION('ref_axis',(1.,0.,0.));
#6031=DIRECTION('center_axis',(0.,1.,0.));
#6032=DIRECTION('ref_axis',(1.,0.,0.));
#6033=DIRECTION('center_axis',(0.,1.,0.));
#6034=DIRECTION('ref_axis',(1.,0.,0.));
#6035=DIRECTION('',(0.,1.,0.));
#6036=DIRECTION('center_axis',(0.,-1.,0.));
#6037=DIRECTION('ref_axis',(1.,0.,0.));
#6038=DIRECTION('center_axis',(0.,1.,0.));
#6039=DIRECTION('ref_axis',(1.,0.,0.));
#6040=DIRECTION('center_axis',(0.,1.,0.));
#6041=DIRECTION('ref_axis',(1.,0.,0.));
#6042=DIRECTION('',(0.,1.,0.));
#6043=DIRECTION('center_axis',(0.,-1.,0.));
#6044=DIRECTION('ref_axis',(1.,0.,0.));
#6045=DIRECTION('center_axis',(0.,1.,0.));
#6046=DIRECTION('ref_axis',(1.,0.,0.));
#6047=DIRECTION('center_axis',(0.,1.,0.));
#6048=DIRECTION('ref_axis',(1.,0.,0.));
#6049=DIRECTION('',(0.,1.,0.));
#6050=DIRECTION('center_axis',(-0.832050294337844,0.,-0.554700196225229));
#6051=DIRECTION('ref_axis',(-0.554700196225229,0.,0.832050294337844));
#6052=DIRECTION('',(0.554700196225229,0.,-0.832050294337844));
#6053=DIRECTION('',(0.,1.,0.));
#6054=DIRECTION('',(-0.554700196225229,0.,0.832050294337844));
#6055=DIRECTION('',(0.,1.,0.));
#6056=DIRECTION('center_axis',(0.,0.,-1.));
#6057=DIRECTION('ref_axis',(-1.,0.,0.));
#6058=DIRECTION('',(1.,0.,0.));
#6059=DIRECTION('',(-1.,0.,0.));
#6060=DIRECTION('',(0.,1.,0.));
#6061=DIRECTION('center_axis',(0.832050294337844,0.,-0.554700196225229));
#6062=DIRECTION('ref_axis',(-0.554700196225229,0.,-0.832050294337844));
#6063=DIRECTION('',(0.554700196225229,0.,0.832050294337844));
#6064=DIRECTION('',(-0.554700196225229,0.,-0.832050294337844));
#6065=DIRECTION('',(0.,1.,0.));
#6066=DIRECTION('center_axis',(1.,0.,0.));
#6067=DIRECTION('ref_axis',(0.,0.,-1.));
#6068=DIRECTION('',(0.,0.,1.));
#6069=DIRECTION('',(0.,0.,-1.));
#6070=DIRECTION('',(0.,1.,0.));
#6071=DIRECTION('center_axis',(0.894427190999916,0.,0.447213595499958));
#6072=DIRECTION('ref_axis',(0.447213595499958,0.,-0.894427190999916));
#6073=DIRECTION('',(-0.447213595499958,0.,0.894427190999916));
#6074=DIRECTION('',(0.447213595499958,0.,-0.894427190999916));
#6075=DIRECTION('',(0.,1.,0.));
#6076=DIRECTION('center_axis',(0.,0.,1.));
#6077=DIRECTION('ref_axis',(1.,0.,0.));
#6078=DIRECTION('',(-1.,0.,0.));
#6079=DIRECTION('',(1.,0.,0.));
#6080=DIRECTION('',(0.,1.,0.));
#6081=DIRECTION('center_axis',(-0.894427190999916,0.,0.447213595499958));
#6082=DIRECTION('ref_axis',(0.447213595499958,0.,0.894427190999916));
#6083=DIRECTION('',(-0.447213595499958,0.,-0.894427190999916));
#6084=DIRECTION('',(0.447213595499958,0.,0.894427190999916));
#6085=DIRECTION('',(0.,1.,0.));
#6086=DIRECTION('center_axis',(-1.,0.,0.));
#6087=DIRECTION('ref_axis',(0.,0.,1.));
#6088=DIRECTION('',(0.,0.,-1.));
#6089=DIRECTION('',(0.,0.,1.));
#6090=DIRECTION('center_axis',(0.,1.,0.));
#6091=DIRECTION('ref_axis',(0.,0.,1.));
#6092=DIRECTION('center_axis',(0.,1.,0.));
#6093=DIRECTION('ref_axis',(1.,0.,0.));
#7559=CARTESIAN_POINT('',(0.,0.,0.));
#7560=CARTESIAN_POINT('Origin',(0.,-2.8,12.));
#7561=CARTESIAN_POINT('',(-2.99903459153175,-2.8,10.7476855351806));
#7562=CARTESIAN_POINT('',(-2.60150387000671,-2.8,10.0520067725117));
#7563=CARTESIAN_POINT('Origin',(-3.5,-2.8,10.));
#7564=CARTESIAN_POINT('',(-2.99903459153175,-2.8,13.2523144648194));
#7565=CARTESIAN_POINT('Origin',(0.,-2.8,12.));
#7566=CARTESIAN_POINT('',(-2.60150387000671,-2.8,13.9479932274883));
#7567=CARTESIAN_POINT('Origin',(-3.5,-2.8,14.));
#7568=CARTESIAN_POINT('',(2.60150387000671,-2.8,13.9479932274883));
#7569=CARTESIAN_POINT('Origin',(0.,-2.8,12.));
#7570=CARTESIAN_POINT('',(2.99903459153175,-2.8,13.2523144648194));
#7571=CARTESIAN_POINT('Origin',(3.5,-2.8,14.));
#7572=CARTESIAN_POINT('',(2.99903459153175,-2.8,10.7476855351806));
#7573=CARTESIAN_POINT('Origin',(0.,-2.8,12.));
#7574=CARTESIAN_POINT('',(2.60150387000671,-2.8,10.0520067725117));
#7575=CARTESIAN_POINT('Origin',(3.5,-2.8,10.));
#7576=CARTESIAN_POINT('Origin',(0.,-2.8,12.));
#7577=CARTESIAN_POINT('',(-1.2,-2.8,12.));
#7578=CARTESIAN_POINT('Origin',(0.,-2.8,12.));
#7579=CARTESIAN_POINT('Origin',(0.,-2.8,12.));
#7580=CARTESIAN_POINT('',(2.99903459153175,-2.5,10.7476855351806));
#7581=CARTESIAN_POINT('',(2.99903459153175,-2.8,10.7476855351806));
#7582=CARTESIAN_POINT('',(2.99903459153175,-2.5,13.2523144648194));
#7583=CARTESIAN_POINT('',(2.99903459153175,-2.8,13.2523144648194));
#7584=CARTESIAN_POINT('Origin',(0.,-2.5,12.));
#7585=CARTESIAN_POINT('Origin',(0.,-2.8,12.));
#7586=CARTESIAN_POINT('',(-2.60150387000671,-2.5,13.9479932274883));
#7587=CARTESIAN_POINT('',(-2.60150387000671,-2.8,13.9479932274883));
#7588=CARTESIAN_POINT('',(2.60150387000671,-2.5,13.9479932274883));
#7589=CARTESIAN_POINT('Origin',(0.,-2.5,12.));
#7590=CARTESIAN_POINT('',(2.60150387000671,-2.8,13.9479932274883));
#7591=CARTESIAN_POINT('Origin',(0.,-2.8,12.));
#7592=CARTESIAN_POINT('',(-2.60150387000671,-2.5,10.0520067725117));
#7593=CARTESIAN_POINT('',(-2.60150387000671,-2.8,10.0520067725117));
#7594=CARTESIAN_POINT('',(2.60150387000671,-2.5,10.0520067725117));
#7595=CARTESIAN_POINT('',(2.60150387000671,-2.8,10.0520067725117));
#7596=CARTESIAN_POINT('Origin',(0.,-2.5,12.));
#7597=CARTESIAN_POINT('Origin',(0.,-2.8,12.));
#7598=CARTESIAN_POINT('',(-1.2,-2.5,12.));
#7599=CARTESIAN_POINT('',(-1.2,-2.8,12.));
#7600=CARTESIAN_POINT('Origin',(0.,-2.5,12.));
#7601=CARTESIAN_POINT('Origin',(0.,-2.8,12.));
#7602=CARTESIAN_POINT('',(-2.99903459153175,-2.5,10.7476855351806));
#7603=CARTESIAN_POINT('',(-2.99903459153175,-2.8,10.7476855351806));
#7604=CARTESIAN_POINT('',(-2.99903459153175,-2.5,13.2523144648194));
#7605=CARTESIAN_POINT('Origin',(0.,-2.5,12.));
#7606=CARTESIAN_POINT('',(-2.99903459153175,-2.8,13.2523144648194));
#7607=CARTESIAN_POINT('Origin',(-3.5,-3.2,10.));
#7608=CARTESIAN_POINT('',(-4.4,-3.1,10.));
#7609=CARTESIAN_POINT('Origin',(-3.5,-3.1,10.));
#7610=CARTESIAN_POINT('',(-4.4,-2.5,10.));
#7611=CARTESIAN_POINT('',(-4.4,-3.2,10.));
#7612=CARTESIAN_POINT('Origin',(-3.5,-2.5,10.));
#7613=CARTESIAN_POINT('Origin',(-3.5,-2.5,10.));
#7614=CARTESIAN_POINT('Origin',(3.5,-3.2,10.));
#7615=CARTESIAN_POINT('',(2.6,-3.1,10.));
#7616=CARTESIAN_POINT('Origin',(3.5,-3.1,10.));
#7617=CARTESIAN_POINT('',(2.6,-2.5,10.));
#7618=CARTESIAN_POINT('',(2.6,-3.2,10.));
#7619=CARTESIAN_POINT('Origin',(3.5,-2.5,10.));
#7620=CARTESIAN_POINT('Origin',(3.5,-2.5,10.));
#7621=CARTESIAN_POINT('Origin',(3.5,-3.2,14.));
#7622=CARTESIAN_POINT('',(2.6,-3.1,14.));
#7623=CARTESIAN_POINT('Origin',(3.5,-3.1,14.));
#7624=CARTESIAN_POINT('',(2.6,-2.5,14.));
#7625=CARTESIAN_POINT('',(2.6,-3.2,14.));
#7626=CARTESIAN_POINT('Origin',(3.5,-2.5,14.));
#7627=CARTESIAN_POINT('Origin',(3.5,-2.5,14.));
#7628=CARTESIAN_POINT('Origin',(0.,-2.5,13.25));
#7629=CARTESIAN_POINT('',(-1.,-2.5,12.));
#7630=CARTESIAN_POINT('Origin',(0.,-2.5,12.));
#7631=CARTESIAN_POINT('Origin',(-3.5,-3.2,14.));
#7632=CARTESIAN_POINT('',(-4.4,-3.1,14.));
#7633=CARTESIAN_POINT('Origin',(-3.5,-3.1,14.));
#7634=CARTESIAN_POINT('',(-4.4,-2.5,14.));
#7635=CARTESIAN_POINT('',(-4.4,-3.2,14.));
#7636=CARTESIAN_POINT('Origin',(-3.5,-2.5,14.));
#7637=CARTESIAN_POINT('Origin',(-3.5,-2.5,14.));
#7638=CARTESIAN_POINT('Origin',(-2.,-3.2,5.));
#7639=CARTESIAN_POINT('',(-2.425,-3.1,5.));
#7640=CARTESIAN_POINT('Origin',(-2.,-3.1,5.));
#7641=CARTESIAN_POINT('',(-2.425,-2.5,5.));
#7642=CARTESIAN_POINT('',(-2.425,-3.2,5.));
#7643=CARTESIAN_POINT('Origin',(-2.,-2.5,5.));
#7644=CARTESIAN_POINT('Origin',(2.,-3.2,5.));
#7645=CARTESIAN_POINT('',(1.575,-3.1,5.));
#7646=CARTESIAN_POINT('Origin',(2.,-3.1,5.));
#7647=CARTESIAN_POINT('',(1.575,-2.5,5.));
#7648=CARTESIAN_POINT('',(1.575,-3.2,5.));
#7649=CARTESIAN_POINT('Origin',(2.,-2.5,5.));
#7650=CARTESIAN_POINT('Origin',(0.,-3.2,20.5));
#7651=CARTESIAN_POINT('',(-0.425,-3.1,20.5));
#7652=CARTESIAN_POINT('Origin',(0.,-3.1,20.5));
#7653=CARTESIAN_POINT('',(-0.425,-2.5,20.5));
#7654=CARTESIAN_POINT('',(-0.425,-3.2,20.5));
#7655=CARTESIAN_POINT('Origin',(0.,-2.5,20.5));
#7656=CARTESIAN_POINT('Origin',(0.,-3.2,12.));
#7657=CARTESIAN_POINT('',(-1.,-3.1,12.));
#7658=CARTESIAN_POINT('Origin',(0.,-3.1,12.));
#7659=CARTESIAN_POINT('',(-1.,-3.2,12.));
#7660=CARTESIAN_POINT('Origin',(-3.,-3.1,4.5));
#7661=CARTESIAN_POINT('',(-6.,-3.1,9.));
#7662=CARTESIAN_POINT('',(-3.,-3.1,4.5));
#7663=CARTESIAN_POINT('',(-6.,-3.1,9.));
#7664=CARTESIAN_POINT('',(-6.,-2.5,9.));
#7665=CARTESIAN_POINT('',(-6.,-3.1,9.));
#7666=CARTESIAN_POINT('',(-3.,-2.5,4.5));
#7667=CARTESIAN_POINT('',(-6.,-2.5,9.));
#7668=CARTESIAN_POINT('',(-3.,-3.1,4.5));
#7669=CARTESIAN_POINT('Origin',(3.,-3.1,4.5));
#7670=CARTESIAN_POINT('',(3.,-3.1,4.5));
#7671=CARTESIAN_POINT('',(-3.,-3.1,4.5));
#7672=CARTESIAN_POINT('',(3.,-2.5,4.5));
#7673=CARTESIAN_POINT('',(-3.,-2.5,4.5));
#7674=CARTESIAN_POINT('',(3.,-3.1,4.5));
#7675=CARTESIAN_POINT('Origin',(6.,-3.1,9.));
#7676=CARTESIAN_POINT('',(6.,-3.1,9.));
#7677=CARTESIAN_POINT('',(3.,-3.1,4.5));
#7678=CARTESIAN_POINT('',(6.,-2.5,9.));
#7679=CARTESIAN_POINT('',(3.,-2.5,4.5));
#7680=CARTESIAN_POINT('',(6.,-3.1,9.));
#7681=CARTESIAN_POINT('Origin',(6.,-3.1,15.));
#7682=CARTESIAN_POINT('',(6.,-3.1,15.));
#7683=CARTESIAN_POINT('',(6.,-3.1,9.));
#7684=CARTESIAN_POINT('',(6.,-2.5,15.));
#7685=CARTESIAN_POINT('',(6.,-2.5,9.));
#7686=CARTESIAN_POINT('',(6.,-3.1,15.));
#7687=CARTESIAN_POINT('Origin',(2.5,-3.1,22.));
#7688=CARTESIAN_POINT('',(2.5,-3.1,22.));
#7689=CARTESIAN_POINT('',(6.,-3.1,15.));
#7690=CARTESIAN_POINT('',(2.5,-2.5,22.));
#7691=CARTESIAN_POINT('',(6.,-2.5,15.));
#7692=CARTESIAN_POINT('',(2.5,-3.1,22.));
#7693=CARTESIAN_POINT('Origin',(-2.5,-3.1,22.));
#7694=CARTESIAN_POINT('',(-2.5,-3.1,22.));
#7695=CARTESIAN_POINT('',(2.5,-3.1,22.));
#7696=CARTESIAN_POINT('',(-2.5,-2.5,22.));
#7697=CARTESIAN_POINT('',(2.5,-2.5,22.));
#7698=CARTESIAN_POINT('',(-2.5,-3.1,22.));
#7699=CARTESIAN_POINT('Origin',(-6.,-3.1,15.));
#7700=CARTESIAN_POINT('',(-6.,-3.1,15.));
#7701=CARTESIAN_POINT('',(-2.5,-3.1,22.));
#7702=CARTESIAN_POINT('',(-6.,-2.5,15.));
#7703=CARTESIAN_POINT('',(-2.5,-2.5,22.));
#7704=CARTESIAN_POINT('',(-6.,-3.1,15.));
#7705=CARTESIAN_POINT('Origin',(-6.,-3.1,9.));
#7706=CARTESIAN_POINT('',(-6.,-3.1,15.));
#7707=CARTESIAN_POINT('',(-6.,-2.5,15.));
#7708=CARTESIAN_POINT('Origin',(0.,-2.5,13.25));
#7709=CARTESIAN_POINT('Origin',(0.,-3.1,13.25));
#9320=UNCERTAINTY_MEASURE_WITH_UNIT(LENGTH_MEASURE(0.001),#9392,
'DISTANCE_ACCURACY_VALUE',
'Maximum model space distance between geometric entities at asserted c
onnectivities');
#9354=UNCERTAINTY_MEASURE_WITH_UNIT(LENGTH_MEASURE(0.001),#9392,
'DISTANCE_ACCURACY_VALUE',
'Maximum model space distance between geometric entities at asserted c
onnectivities');
#9357=(
GEOMETRIC_REPRESENTATION_CONTEXT(3)
GLOBAL_UNCERTAINTY_ASSIGNED_CONTEXT((#9320))
GLOBAL_UNIT_ASSIGNED_CONTEXT((#9392,#9394,#9395))
REPRESENTATION_CONTEXT('','3D')
);
#9391=(
GEOMETRIC_REPRESENTATION_CONTEXT(3)
GLOBAL_UNCERTAINTY_ASSIGNED_CONTEXT((#9354))
GLOBAL_UNIT_ASSIGNED_CONTEXT((#9392,#9394,#9395))
REPRESENTATION_CONTEXT('','3D')
);
#9392=(
LENGTH_UNIT()
NAMED_UNIT(*)
SI_UNIT(.CENTI.,.METRE.)
);
#9394=(
NAMED_UNIT(*)
PLANE_ANGLE_UNIT()
SI_UNIT($,.RADIAN.)
);
#9395=(
NAMED_UNIT(*)
SI_UNIT($,.STERADIAN.)
SOLID_ANGLE_UNIT()
);
#9398=SHAPE_DEFINITION_REPRESENTATION(#9434,#9522);
#9434=PRODUCT_DEFINITION_SHAPE('',$,#9559);
#9522=SHAPE_REPRESENTATION('',(#5261),#9357);
#9556=PRODUCT_DEFINITION_CONTEXT('part definition',#9666,'design');
#9559=PRODUCT_DEFINITION('Side plate','Side plate',#9595,#9556);
#9595=PRODUCT_DEFINITION_FORMATION('',$,#9670);
#9666=APPLICATION_CONTEXT(
'Core Data for Automotive Mechanical Design Process');
#9667=PRODUCT_CONTEXT('part definition',#9666,'mechanical');
#9670=PRODUCT('Side plate','Side plate','Side plate',(#9667));
#9746=COLOUR_RGB('Sky Blue',0.24,0.69,0.87);
#9747=FILL_AREA_STYLE_COLOUR('',#9746);
#9748=FILL_AREA_STYLE('',(#9747));
#9749=SURFACE_STYLE_FILL_AREA(#9748);
#9750=SURFACE_SIDE_STYLE('',(#9749));
#9751=SURFACE_STYLE_USAGE(.BOTH.,#9750);
#9752=PRESENTATION_STYLE_ASSIGNMENT((#9751));
ENDSEC;
END-ISO-10303-21;
